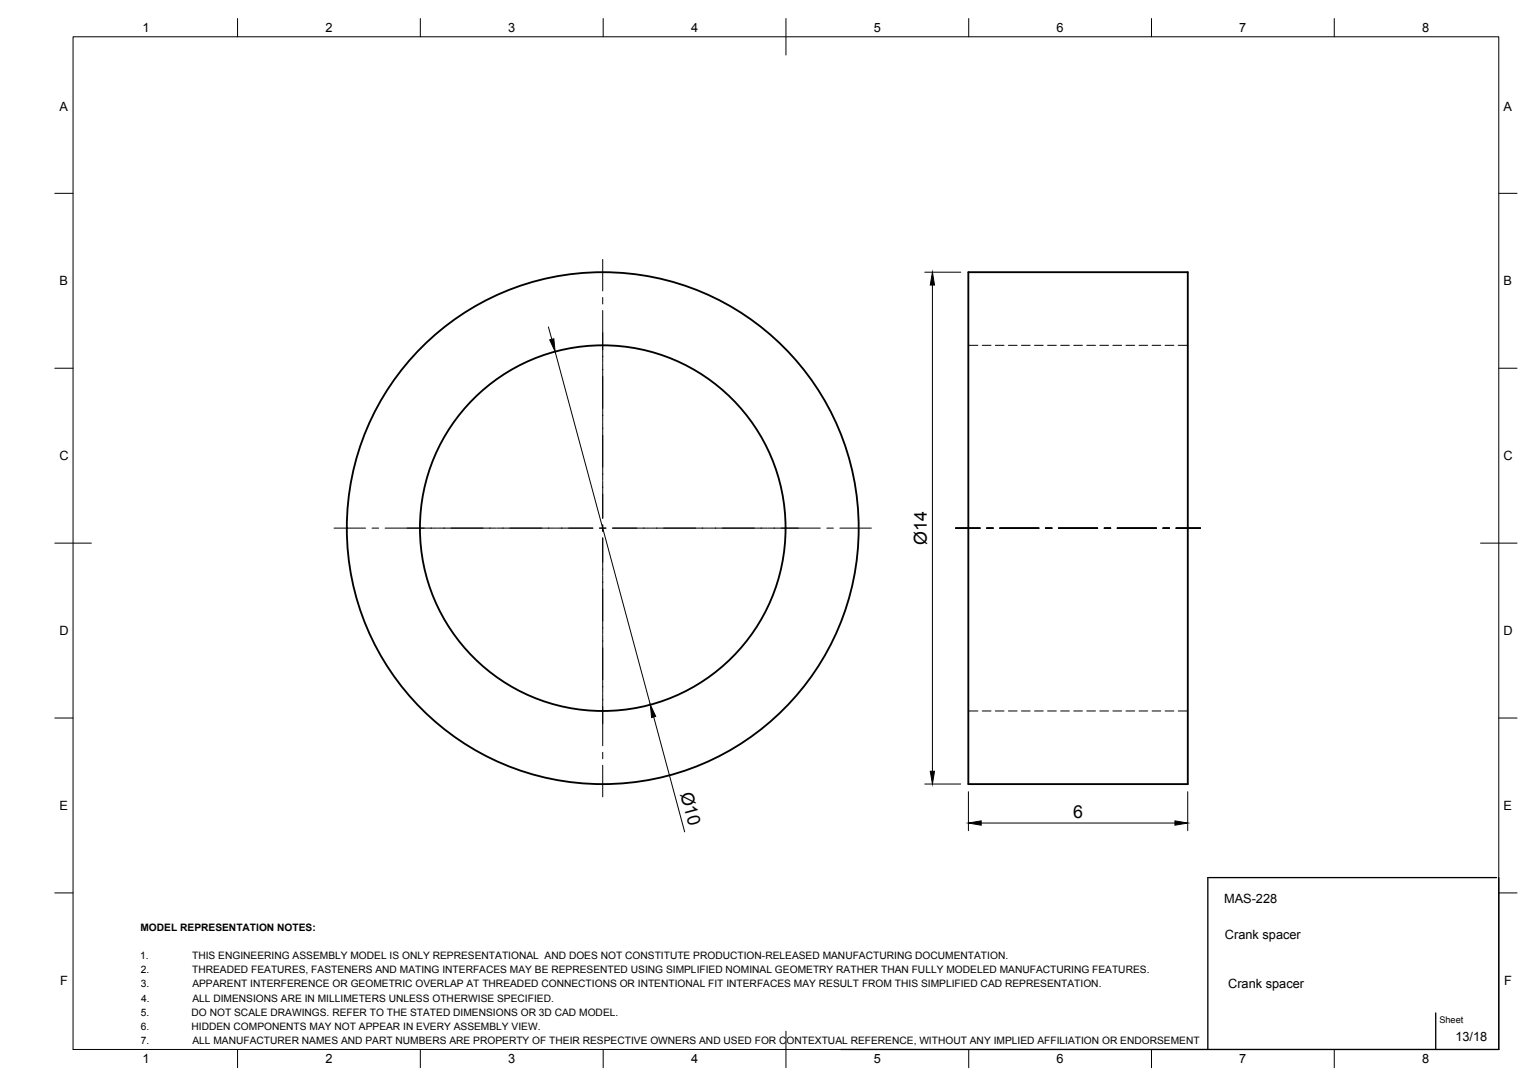
ISO-10303-21;
HEADER;
/* Generated by software containing ST-Developer
 * from STEP Tools, Inc. (www.steptools.com) 
 */

FILE_DESCRIPTION(
/* description */ ('Independent Peaucellier-Lipkin straight-line linkage. Radius arms 100
 mm, inversion-cell links 60 mm, crank radius and fixed-pivot spacing 
32 mm. Inversion constant 6400 mm squared, nominal output straight lin
e X=100 mm. Overhead bearing bridge clears the layered moving links. N
o accuracy or load rating assigned.'),
/* implementation_level */ '2;1');

FILE_NAME(
/* name */ 'Crank spacer.step',
/* time_stamp */ '2026-11-09T18:06:16-08:00',
/* author */ (''),
/* organization */ (''),
/* preprocessor_version */ 'ST-DEVELOPER v20.2',
/* originating_system */ 'Autodesk Translation Framework v15.17.0.0',
/* authorisation */ '');

FILE_SCHEMA (('AUTOMOTIVE_DESIGN { 1 0 10303 214 3 1 1 }'));
ENDSEC;

DATA;
#10=MECHANICAL_DESIGN_GEOMETRIC_PRESENTATION_REPRESENTATION('',(#291),#3581);
#257=SHAPE_REPRESENTATION_RELATIONSHIP('SRR','None',#3691,#274);
#274=ADVANCED_BREP_SHAPE_REPRESENTATION('',(#308),#3573);
#291=STYLED_ITEM('',(#3783),#308);
#308=MANIFOLD_SOLID_BREP('Body1',#1877);
#348=FACE_BOUND('',#638,.T.);
#349=FACE_BOUND('',#640,.T.);
#402=PLANE('',#2215);
#403=PLANE('',#2216);
#492=FACE_OUTER_BOUND('',#635,.T.);
#493=FACE_OUTER_BOUND('',#636,.T.);
#494=FACE_OUTER_BOUND('',#637,.T.);
#495=FACE_OUTER_BOUND('',#639,.T.);
#635=EDGE_LOOP('',(#1574,#1575,#1576,#1577));
#636=EDGE_LOOP('',(#1578,#1579,#1580,#1581));
#637=EDGE_LOOP('',(#1582));
#638=EDGE_LOOP('',(#1583));
#639=EDGE_LOOP('',(#1584));
#640=EDGE_LOOP('',(#1585));
#766=LINE('',#3326,#864);
#767=LINE('',#3332,#865);
#864=VECTOR('',#2706,5.);
#865=VECTOR('',#2713,7.);
#949=CIRCLE('',#2210,5.);
#950=CIRCLE('',#2211,5.);
#951=CIRCLE('',#2213,7.);
#952=CIRCLE('',#2214,7.);
#1075=VERTEX_POINT('',#3323);
#1076=VERTEX_POINT('',#3325);
#1077=VERTEX_POINT('',#3329);
#1078=VERTEX_POINT('',#3331);
#1249=EDGE_CURVE('',#1075,#1075,#949,.T.);
#1250=EDGE_CURVE('',#1075,#1076,#766,.T.);
#1251=EDGE_CURVE('',#1076,#1076,#950,.T.);
#1252=EDGE_CURVE('',#1077,#1077,#951,.T.);
#1253=EDGE_CURVE('',#1077,#1078,#767,.T.);
#1254=EDGE_CURVE('',#1078,#1078,#952,.T.);
#1574=ORIENTED_EDGE('',*,*,#1249,.F.);
#1575=ORIENTED_EDGE('',*,*,#1250,.T.);
#1576=ORIENTED_EDGE('',*,*,#1251,.T.);
#1577=ORIENTED_EDGE('',*,*,#1250,.F.);
#1578=ORIENTED_EDGE('',*,*,#1252,.F.);
#1579=ORIENTED_EDGE('',*,*,#1253,.T.);
#1580=ORIENTED_EDGE('',*,*,#1254,.T.);
#1581=ORIENTED_EDGE('',*,*,#1253,.F.);
#1582=ORIENTED_EDGE('',*,*,#1252,.T.);
#1583=ORIENTED_EDGE('',*,*,#1249,.T.);
#1584=ORIENTED_EDGE('',*,*,#1254,.F.);
#1585=ORIENTED_EDGE('',*,*,#1251,.F.);
#1737=CYLINDRICAL_SURFACE('',#2209,5.);
#1738=CYLINDRICAL_SURFACE('',#2212,7.);
#1824=ADVANCED_FACE('',(#492),#1737,.F.);
#1825=ADVANCED_FACE('',(#493),#1738,.T.);
#1826=ADVANCED_FACE('',(#494,#348),#402,.T.);
#1827=ADVANCED_FACE('',(#495,#349),#403,.F.);
#1877=CLOSED_SHELL('',(#1824,#1825,#1826,#1827));
#2208=AXIS2_PLACEMENT_3D('',#3321,#2700,#2701);
#2209=AXIS2_PLACEMENT_3D('',#3322,#2702,#2703);
#2210=AXIS2_PLACEMENT_3D('',#3324,#2704,#2705);
#2211=AXIS2_PLACEMENT_3D('',#3327,#2707,#2708);
#2212=AXIS2_PLACEMENT_3D('',#3328,#2709,#2710);
#2213=AXIS2_PLACEMENT_3D('',#3330,#2711,#2712);
#2214=AXIS2_PLACEMENT_3D('',#3333,#2714,#2715);
#2215=AXIS2_PLACEMENT_3D('',#3334,#2716,#2717);
#2216=AXIS2_PLACEMENT_3D('',#3335,#2718,#2719);
#2700=DIRECTION('axis',(0.,0.,1.));
#2701=DIRECTION('refdir',(1.,0.,0.));
#2702=DIRECTION('center_axis',(0.,0.,1.));
#2703=DIRECTION('ref_axis',(1.,0.,0.));
#2704=DIRECTION('center_axis',(0.,0.,-1.));
#2705=DIRECTION('ref_axis',(1.,0.,0.));
#2706=DIRECTION('',(0.,0.,-1.));
#2707=DIRECTION('center_axis',(0.,0.,-1.));
#2708=DIRECTION('ref_axis',(1.,0.,0.));
#2709=DIRECTION('center_axis',(0.,0.,1.));
#2710=DIRECTION('ref_axis',(1.,0.,0.));
#2711=DIRECTION('center_axis',(0.,0.,1.));
#2712=DIRECTION('ref_axis',(1.,0.,0.));
#2713=DIRECTION('',(0.,0.,-1.));
#2714=DIRECTION('center_axis',(0.,0.,1.));
#2715=DIRECTION('ref_axis',(1.,0.,0.));
#2716=DIRECTION('center_axis',(0.,0.,1.));
#2717=DIRECTION('ref_axis',(1.,0.,0.));
#2718=DIRECTION('center_axis',(0.,0.,1.));
#2719=DIRECTION('ref_axis',(1.,0.,0.));
#3321=CARTESIAN_POINT('',(0.,0.,0.));
#3322=CARTESIAN_POINT('Origin',(0.,0.,0.));
#3323=CARTESIAN_POINT('',(-5.,-6.12323399573677E-16,6.));
#3324=CARTESIAN_POINT('Origin',(0.,0.,6.));
#3325=CARTESIAN_POINT('',(-5.,-6.12323399573677E-16,0.));
#3326=CARTESIAN_POINT('',(-5.,-6.12323399573677E-16,0.));
#3327=CARTESIAN_POINT('Origin',(0.,0.,0.));
#3328=CARTESIAN_POINT('Origin',(0.,0.,0.));
#3329=CARTESIAN_POINT('',(-7.,-8.57252759403147E-16,6.));
#3330=CARTESIAN_POINT('Origin',(0.,0.,6.));
#3331=CARTESIAN_POINT('',(-7.,-8.57252759403147E-16,0.));
#3332=CARTESIAN_POINT('',(-7.,-8.57252759403147E-16,0.));
#3333=CARTESIAN_POINT('Origin',(0.,0.,0.));
#3334=CARTESIAN_POINT('Origin',(0.,0.,6.));
#3335=CARTESIAN_POINT('Origin',(0.,0.,0.));
#3554=UNCERTAINTY_MEASURE_WITH_UNIT(LENGTH_MEASURE(0.01),#3582,
'DISTANCE_ACCURACY_VALUE',
'Maximum model space distance between geometric entities at asserted c
onnectivities');
#3562=UNCERTAINTY_MEASURE_WITH_UNIT(LENGTH_MEASURE(0.01),#3582,
'DISTANCE_ACCURACY_VALUE',
'Maximum model space distance between geometric entities at asserted c
onnectivities');
#3573=(
GEOMETRIC_REPRESENTATION_CONTEXT(3)
GLOBAL_UNCERTAINTY_ASSIGNED_CONTEXT((#3554))
GLOBAL_UNIT_ASSIGNED_CONTEXT((#3582,#3584,#3585))
REPRESENTATION_CONTEXT('','3D')
);
#3581=(
GEOMETRIC_REPRESENTATION_CONTEXT(3)
GLOBAL_UNCERTAINTY_ASSIGNED_CONTEXT((#3562))
GLOBAL_UNIT_ASSIGNED_CONTEXT((#3582,#3584,#3585))
REPRESENTATION_CONTEXT('','3D')
);
#3582=(
LENGTH_UNIT()
NAMED_UNIT(*)
SI_UNIT(.MILLI.,.METRE.)
);
#3584=(
NAMED_UNIT(*)
PLANE_ANGLE_UNIT()
SI_UNIT($,.RADIAN.)
);
#3585=(
NAMED_UNIT(*)
SI_UNIT($,.STERADIAN.)
SOLID_ANGLE_UNIT()
);
#3596=SHAPE_DEFINITION_REPRESENTATION(#3614,#3691);
#3614=PRODUCT_DEFINITION_SHAPE('',$,#3710);
#3691=SHAPE_REPRESENTATION('',(#2208),#3573);
#3699=PRODUCT_DEFINITION_CONTEXT('part definition',#3755,'design');
#3710=PRODUCT_DEFINITION('Crank spacer','Crank spacer',#3728,#3699);
#3728=PRODUCT_DEFINITION_FORMATION('',$,#3767);
#3755=APPLICATION_CONTEXT(
'Core Data for Automotive Mechanical Design Process');
#3756=PRODUCT_CONTEXT('part definition',#3755,'mechanical');
#3767=PRODUCT('Crank spacer','Crank spacer','Crank spacer',(#3756));
#3783=PRESENTATION_STYLE_ASSIGNMENT((#3796));
#3796=SURFACE_STYLE_USAGE(.BOTH.,#3809);
#3809=SURFACE_SIDE_STYLE('',(#3822));
#3822=SURFACE_STYLE_FILL_AREA(#3835);
#3835=FILL_AREA_STYLE('Spacer light gray',(#3848));
#3848=FILL_AREA_STYLE_COLOUR('Spacer light gray',#3861);
#3861=COLOUR_RGB('Spacer light gray',0.725490196078431,0.752941176470588,
0.792156862745098);
ENDSEC;
END-ISO-10303-21;
